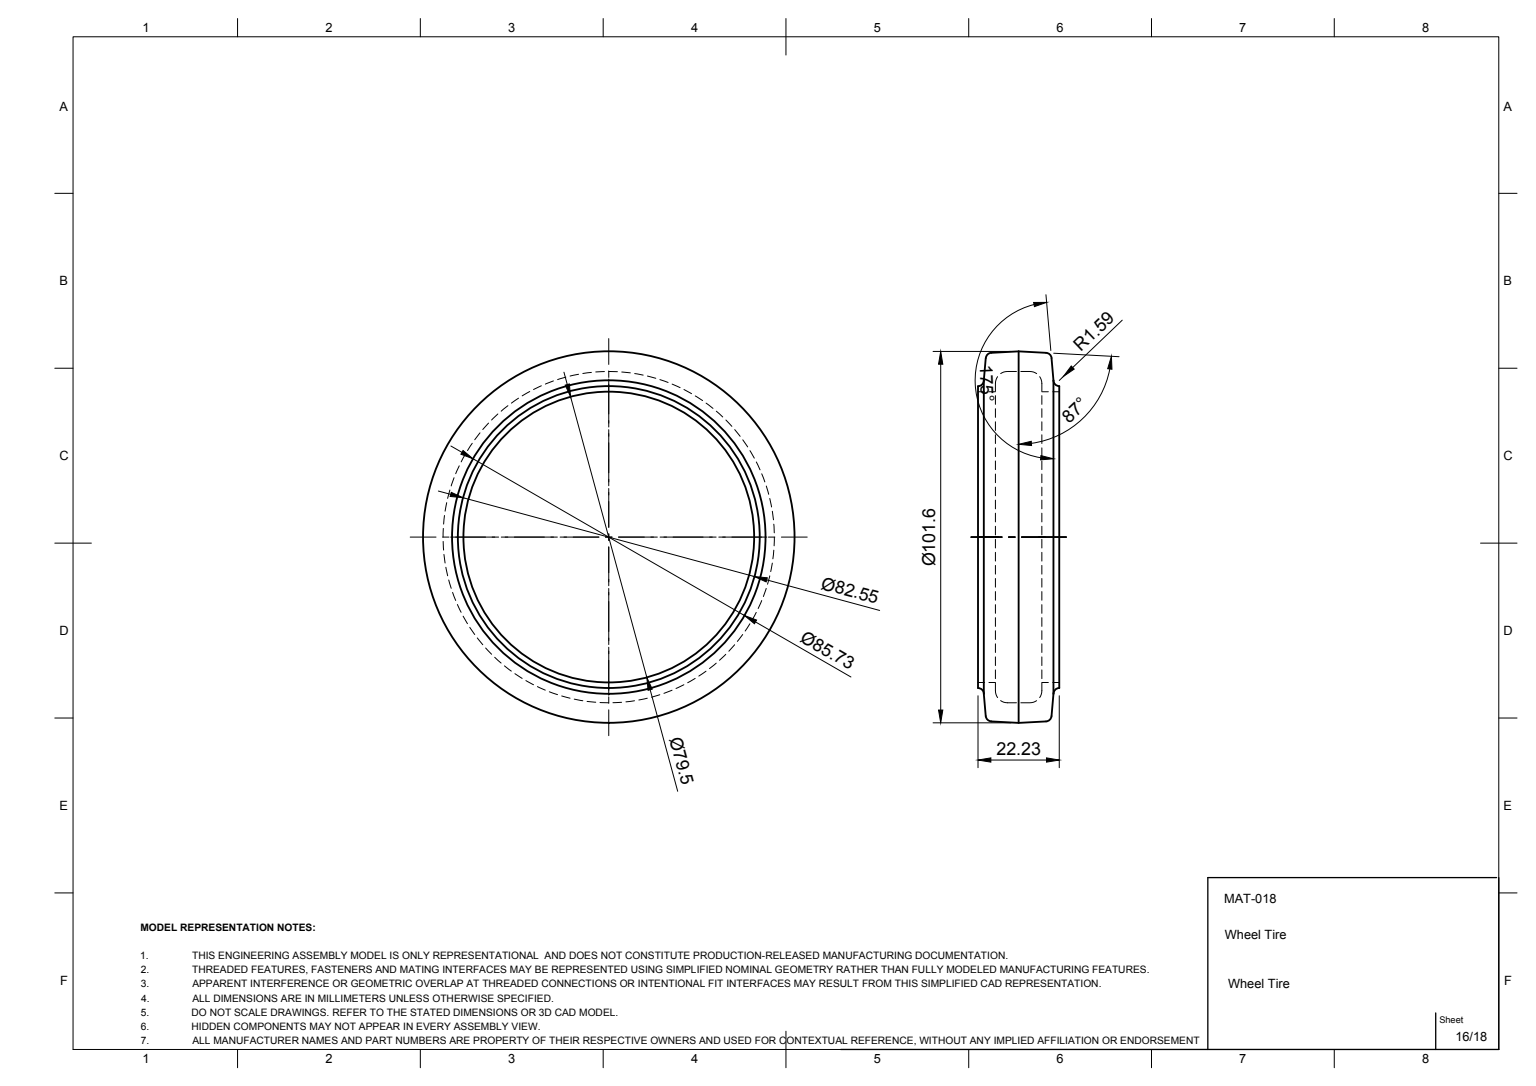
ISO-10303-21;
HEADER;
/* Generated by software containing ST-Developer
 * from STEP Tools, Inc. (www.steptools.com) 
 */

FILE_DESCRIPTION(
/* description */ ('STEP AP214'),
/* implementation_level */ '2;1');

FILE_NAME(
/* name */ 'Wheel Tire.step',
/* time_stamp */ '2026-11-14T06:16:09-08:00',
/* author */ (''),
/* organization */ (''),
/* preprocessor_version */ 'ST-DEVELOPER v20.2',
/* originating_system */ 'Autodesk Translation Framework v15.17.0.0',
/* authorisation */ '');

FILE_SCHEMA (('AUTOMOTIVE_DESIGN { 1 0 10303 214 3 1 1 }'));
ENDSEC;

DATA;
#10=MECHANICAL_DESIGN_GEOMETRIC_PRESENTATION_REPRESENTATION('',(#360),#18006);
#147=CONICAL_SURFACE('',#10793,42.8625,1.48352986419518);
#148=CONICAL_SURFACE('',#10800,50.4073015581831,0.0523598775598306);
#149=CONICAL_SURFACE('',#10803,50.8,0.0523598775598286);
#150=CONICAL_SURFACE('',#10808,48.9603369133721,1.48352986419518);
#262=TOROIDAL_SURFACE('',#10776,42.00525,3.302);
#263=TOROIDAL_SURFACE('',#10782,42.00525,3.302);
#264=TOROIDAL_SURFACE('',#10788,42.8625,1.5875);
#265=TOROIDAL_SURFACE('',#10796,48.8219771717602,1.5875);
#266=TOROIDAL_SURFACE('',#10805,48.8219771717602,1.5875);
#267=TOROIDAL_SURFACE('',#10810,42.8625,1.5875);
#328=SHAPE_REPRESENTATION_RELATIONSHIP('SRR','None',#18086,#344);
#344=ADVANCED_BREP_SHAPE_REPRESENTATION('',(#376),#18003);
#360=STYLED_ITEM('',(#18172),#376);
#376=MANIFOLD_SOLID_BREP('Body1',#9569);
#494=FACE_BOUND('',#2095,.T.);
#495=FACE_BOUND('',#2097,.T.);
#496=FACE_BOUND('',#2099,.T.);
#497=FACE_BOUND('',#2101,.T.);
#833=PLANE('',#10813);
#834=PLANE('',#10814);
#835=PLANE('',#10815);
#836=PLANE('',#10816);
#1390=FACE_OUTER_BOUND('',#2081,.T.);
#1391=FACE_OUTER_BOUND('',#2082,.T.);
#1392=FACE_OUTER_BOUND('',#2083,.T.);
#1393=FACE_OUTER_BOUND('',#2084,.T.);
#1394=FACE_OUTER_BOUND('',#2085,.T.);
#1395=FACE_OUTER_BOUND('',#2086,.T.);
#1396=FACE_OUTER_BOUND('',#2087,.T.);
#1397=FACE_OUTER_BOUND('',#2088,.T.);
#1398=FACE_OUTER_BOUND('',#2089,.T.);
#1399=FACE_OUTER_BOUND('',#2090,.T.);
#1400=FACE_OUTER_BOUND('',#2091,.T.);
#1401=FACE_OUTER_BOUND('',#2092,.T.);
#1402=FACE_OUTER_BOUND('',#2093,.T.);
#1403=FACE_OUTER_BOUND('',#2094,.T.);
#1404=FACE_OUTER_BOUND('',#2096,.T.);
#1405=FACE_OUTER_BOUND('',#2098,.T.);
#1406=FACE_OUTER_BOUND('',#2100,.T.);
#2081=EDGE_LOOP('',(#8706,#8707,#8708,#8709));
#2082=EDGE_LOOP('',(#8710,#8711,#8712,#8713));
#2083=EDGE_LOOP('',(#8714,#8715,#8716,#8717));
#2084=EDGE_LOOP('',(#8718,#8719,#8720,#8721));
#2085=EDGE_LOOP('',(#8722,#8723,#8724,#8725));
#2086=EDGE_LOOP('',(#8726,#8727,#8728,#8729,#8730));
#2087=EDGE_LOOP('',(#8731,#8732,#8733,#8734,#8735,#8736));
#2088=EDGE_LOOP('',(#8737,#8738,#8739,#8740,#8741,#8742));
#2089=EDGE_LOOP('',(#8743,#8744,#8745,#8746,#8747,#8748));
#2090=EDGE_LOOP('',(#8749,#8750,#8751,#8752,#8753));
#2091=EDGE_LOOP('',(#8754,#8755,#8756,#8757));
#2092=EDGE_LOOP('',(#8758,#8759,#8760,#8761));
#2093=EDGE_LOOP('',(#8762,#8763,#8764,#8765));
#2094=EDGE_LOOP('',(#8766));
#2095=EDGE_LOOP('',(#8767));
#2096=EDGE_LOOP('',(#8768));
#2097=EDGE_LOOP('',(#8769));
#2098=EDGE_LOOP('',(#8770));
#2099=EDGE_LOOP('',(#8771));
#2100=EDGE_LOOP('',(#8772));
#2101=EDGE_LOOP('',(#8773));
#2827=LINE('',#17838,#3551);
#2828=LINE('',#17848,#3552);
#2829=LINE('',#17858,#3553);
#2830=LINE('',#17872,#3554);
#2831=LINE('',#17884,#3555);
#2832=LINE('',#17888,#3556);
#2833=LINE('',#17896,#3557);
#3551=VECTOR('',#13624,39.751);
#3552=VECTOR('',#13637,45.30725);
#3553=VECTOR('',#13650,39.751);
#3554=VECTOR('',#13667,42.8625);
#3555=VECTOR('',#13682,50.4073015581831);
#3556=VECTOR('',#13687,50.8);
#3557=VECTOR('',#13698,48.9603369133721);
#3975=CIRCLE('',#10774,39.751);
#3976=CIRCLE('',#10775,39.751);
#3977=CIRCLE('',#10777,42.00525);
#3978=CIRCLE('',#10778,3.302);
#3979=CIRCLE('',#10779,45.30725);
#3980=CIRCLE('',#10781,45.30725);
#3981=CIRCLE('',#10783,3.302);
#3982=CIRCLE('',#10784,42.00525);
#3983=CIRCLE('',#10786,39.751);
#3984=CIRCLE('',#10787,39.751);
#3985=CIRCLE('',#10789,41.275);
#3986=CIRCLE('',#10790,1.5875);
#3987=CIRCLE('',#10791,42.8625);
#3988=CIRCLE('',#10792,42.8625);
#3989=CIRCLE('',#10794,48.9603369133721);
#3990=CIRCLE('',#10795,48.9603369133721);
#3991=CIRCLE('',#10797,1.5875);
#3992=CIRCLE('',#10798,50.4073015581831);
#3993=CIRCLE('',#10799,50.4073015581831);
#3994=CIRCLE('',#10801,50.8);
#3995=CIRCLE('',#10802,50.8);
#3996=CIRCLE('',#10804,50.4073015581831);
#3997=CIRCLE('',#10806,1.5875);
#3998=CIRCLE('',#10807,48.9603369133721);
#3999=CIRCLE('',#10809,42.8625);
#4000=CIRCLE('',#10811,1.5875);
#4001=CIRCLE('',#10812,41.275);
#4792=VERTEX_POINT('',#17835);
#4793=VERTEX_POINT('',#17837);
#4794=VERTEX_POINT('',#17841);
#4795=VERTEX_POINT('',#17843);
#4796=VERTEX_POINT('',#17847);
#4797=VERTEX_POINT('',#17851);
#4798=VERTEX_POINT('',#17855);
#4799=VERTEX_POINT('',#17857);
#4800=VERTEX_POINT('',#17861);
#4801=VERTEX_POINT('',#17863);
#4802=VERTEX_POINT('',#17865);
#4803=VERTEX_POINT('',#17869);
#4804=VERTEX_POINT('',#17870);
#4805=VERTEX_POINT('',#17875);
#4806=VERTEX_POINT('',#17877);
#4807=VERTEX_POINT('',#17881);
#4808=VERTEX_POINT('',#17882);
#4809=VERTEX_POINT('',#17887);
#4810=VERTEX_POINT('',#17891);
#4811=VERTEX_POINT('',#17895);
#4812=VERTEX_POINT('',#17899);
#6101=EDGE_CURVE('',#4792,#4792,#3975,.T.);
#6102=EDGE_CURVE('',#4792,#4793,#2827,.T.);
#6103=EDGE_CURVE('',#4793,#4793,#3976,.T.);
#6104=EDGE_CURVE('',#4794,#4794,#3977,.T.);
#6105=EDGE_CURVE('',#4794,#4795,#3978,.T.);
#6106=EDGE_CURVE('',#4795,#4795,#3979,.T.);
#6107=EDGE_CURVE('',#4795,#4796,#2828,.T.);
#6108=EDGE_CURVE('',#4796,#4796,#3980,.T.);
#6109=EDGE_CURVE('',#4796,#4797,#3981,.T.);
#6110=EDGE_CURVE('',#4797,#4797,#3982,.T.);
#6111=EDGE_CURVE('',#4798,#4798,#3983,.T.);
#6112=EDGE_CURVE('',#4798,#4799,#2829,.T.);
#6113=EDGE_CURVE('',#4799,#4799,#3984,.T.);
#6114=EDGE_CURVE('',#4800,#4800,#3985,.T.);
#6115=EDGE_CURVE('',#4800,#4801,#3986,.T.);
#6116=EDGE_CURVE('',#4801,#4802,#3987,.T.);
#6117=EDGE_CURVE('',#4802,#4801,#3988,.T.);
#6118=EDGE_CURVE('',#4803,#4804,#3989,.T.);
#6119=EDGE_CURVE('',#4804,#4802,#2830,.T.);
#6120=EDGE_CURVE('',#4804,#4803,#3990,.T.);
#6121=EDGE_CURVE('',#4803,#4805,#3991,.T.);
#6122=EDGE_CURVE('',#4805,#4806,#3992,.T.);
#6123=EDGE_CURVE('',#4806,#4805,#3993,.T.);
#6124=EDGE_CURVE('',#4807,#4808,#3994,.T.);
#6125=EDGE_CURVE('',#4808,#4806,#2831,.T.);
#6126=EDGE_CURVE('',#4808,#4807,#3995,.T.);
#6127=EDGE_CURVE('',#4807,#4809,#2832,.T.);
#6128=EDGE_CURVE('',#4809,#4809,#3996,.T.);
#6129=EDGE_CURVE('',#4809,#4810,#3997,.T.);
#6130=EDGE_CURVE('',#4810,#4810,#3998,.T.);
#6131=EDGE_CURVE('',#4810,#4811,#2833,.T.);
#6132=EDGE_CURVE('',#4811,#4811,#3999,.T.);
#6133=EDGE_CURVE('',#4811,#4812,#4000,.T.);
#6134=EDGE_CURVE('',#4812,#4812,#4001,.T.);
#8706=ORIENTED_EDGE('',*,*,#6101,.F.);
#8707=ORIENTED_EDGE('',*,*,#6102,.T.);
#8708=ORIENTED_EDGE('',*,*,#6103,.T.);
#8709=ORIENTED_EDGE('',*,*,#6102,.F.);
#8710=ORIENTED_EDGE('',*,*,#6104,.F.);
#8711=ORIENTED_EDGE('',*,*,#6105,.T.);
#8712=ORIENTED_EDGE('',*,*,#6106,.T.);
#8713=ORIENTED_EDGE('',*,*,#6105,.F.);
#8714=ORIENTED_EDGE('',*,*,#6106,.F.);
#8715=ORIENTED_EDGE('',*,*,#6107,.T.);
#8716=ORIENTED_EDGE('',*,*,#6108,.T.);
#8717=ORIENTED_EDGE('',*,*,#6107,.F.);
#8718=ORIENTED_EDGE('',*,*,#6108,.F.);
#8719=ORIENTED_EDGE('',*,*,#6109,.T.);
#8720=ORIENTED_EDGE('',*,*,#6110,.T.);
#8721=ORIENTED_EDGE('',*,*,#6109,.F.);
#8722=ORIENTED_EDGE('',*,*,#6111,.F.);
#8723=ORIENTED_EDGE('',*,*,#6112,.T.);
#8724=ORIENTED_EDGE('',*,*,#6113,.T.);
#8725=ORIENTED_EDGE('',*,*,#6112,.F.);
#8726=ORIENTED_EDGE('',*,*,#6114,.F.);
#8727=ORIENTED_EDGE('',*,*,#6115,.T.);
#8728=ORIENTED_EDGE('',*,*,#6116,.T.);
#8729=ORIENTED_EDGE('',*,*,#6117,.T.);
#8730=ORIENTED_EDGE('',*,*,#6115,.F.);
#8731=ORIENTED_EDGE('',*,*,#6118,.T.);
#8732=ORIENTED_EDGE('',*,*,#6119,.T.);
#8733=ORIENTED_EDGE('',*,*,#6116,.F.);
#8734=ORIENTED_EDGE('',*,*,#6117,.F.);
#8735=ORIENTED_EDGE('',*,*,#6119,.F.);
#8736=ORIENTED_EDGE('',*,*,#6120,.T.);
#8737=ORIENTED_EDGE('',*,*,#6118,.F.);
#8738=ORIENTED_EDGE('',*,*,#6121,.T.);
#8739=ORIENTED_EDGE('',*,*,#6122,.T.);
#8740=ORIENTED_EDGE('',*,*,#6123,.T.);
#8741=ORIENTED_EDGE('',*,*,#6121,.F.);
#8742=ORIENTED_EDGE('',*,*,#6120,.F.);
#8743=ORIENTED_EDGE('',*,*,#6124,.T.);
#8744=ORIENTED_EDGE('',*,*,#6125,.T.);
#8745=ORIENTED_EDGE('',*,*,#6122,.F.);
#8746=ORIENTED_EDGE('',*,*,#6123,.F.);
#8747=ORIENTED_EDGE('',*,*,#6125,.F.);
#8748=ORIENTED_EDGE('',*,*,#6126,.T.);
#8749=ORIENTED_EDGE('',*,*,#6124,.F.);
#8750=ORIENTED_EDGE('',*,*,#6127,.T.);
#8751=ORIENTED_EDGE('',*,*,#6128,.T.);
#8752=ORIENTED_EDGE('',*,*,#6127,.F.);
#8753=ORIENTED_EDGE('',*,*,#6126,.F.);
#8754=ORIENTED_EDGE('',*,*,#6128,.F.);
#8755=ORIENTED_EDGE('',*,*,#6129,.T.);
#8756=ORIENTED_EDGE('',*,*,#6130,.T.);
#8757=ORIENTED_EDGE('',*,*,#6129,.F.);
#8758=ORIENTED_EDGE('',*,*,#6130,.F.);
#8759=ORIENTED_EDGE('',*,*,#6131,.T.);
#8760=ORIENTED_EDGE('',*,*,#6132,.T.);
#8761=ORIENTED_EDGE('',*,*,#6131,.F.);
#8762=ORIENTED_EDGE('',*,*,#6132,.F.);
#8763=ORIENTED_EDGE('',*,*,#6133,.T.);
#8764=ORIENTED_EDGE('',*,*,#6134,.T.);
#8765=ORIENTED_EDGE('',*,*,#6133,.F.);
#8766=ORIENTED_EDGE('',*,*,#6114,.T.);
#8767=ORIENTED_EDGE('',*,*,#6113,.F.);
#8768=ORIENTED_EDGE('',*,*,#6110,.F.);
#8769=ORIENTED_EDGE('',*,*,#6111,.T.);
#8770=ORIENTED_EDGE('',*,*,#6104,.T.);
#8771=ORIENTED_EDGE('',*,*,#6103,.F.);
#8772=ORIENTED_EDGE('',*,*,#6134,.F.);
#8773=ORIENTED_EDGE('',*,*,#6101,.T.);
#8973=CYLINDRICAL_SURFACE('',#10773,39.751);
#8974=CYLINDRICAL_SURFACE('',#10780,45.30725);
#8975=CYLINDRICAL_SURFACE('',#10785,39.751);
#9529=ADVANCED_FACE('',(#1390),#8973,.F.);
#9530=ADVANCED_FACE('',(#1391),#262,.F.);
#9531=ADVANCED_FACE('',(#1392),#8974,.F.);
#9532=ADVANCED_FACE('',(#1393),#263,.F.);
#9533=ADVANCED_FACE('',(#1394),#8975,.F.);
#9534=ADVANCED_FACE('',(#1395),#264,.F.);
#9535=ADVANCED_FACE('',(#1396),#147,.T.);
#9536=ADVANCED_FACE('',(#1397),#265,.T.);
#9537=ADVANCED_FACE('',(#1398),#148,.T.);
#9538=ADVANCED_FACE('',(#1399),#149,.T.);
#9539=ADVANCED_FACE('',(#1400),#266,.T.);
#9540=ADVANCED_FACE('',(#1401),#150,.T.);
#9541=ADVANCED_FACE('',(#1402),#267,.F.);
#9542=ADVANCED_FACE('',(#1403,#494),#833,.T.);
#9543=ADVANCED_FACE('',(#1404,#495),#834,.T.);
#9544=ADVANCED_FACE('',(#1405,#496),#835,.T.);
#9545=ADVANCED_FACE('',(#1406,#497),#836,.T.);
#9569=CLOSED_SHELL('',(#9529,#9530,#9531,#9532,#9533,#9534,#9535,#9536,
#9537,#9538,#9539,#9540,#9541,#9542,#9543,#9544,#9545));
#10772=AXIS2_PLACEMENT_3D('',#17833,#13618,#13619);
#10773=AXIS2_PLACEMENT_3D('',#17834,#13620,#13621);
#10774=AXIS2_PLACEMENT_3D('',#17836,#13622,#13623);
#10775=AXIS2_PLACEMENT_3D('',#17839,#13625,#13626);
#10776=AXIS2_PLACEMENT_3D('',#17840,#13627,#13628);
#10777=AXIS2_PLACEMENT_3D('',#17842,#13629,#13630);
#10778=AXIS2_PLACEMENT_3D('',#17844,#13631,#13632);
#10779=AXIS2_PLACEMENT_3D('',#17845,#13633,#13634);
#10780=AXIS2_PLACEMENT_3D('',#17846,#13635,#13636);
#10781=AXIS2_PLACEMENT_3D('',#17849,#13638,#13639);
#10782=AXIS2_PLACEMENT_3D('',#17850,#13640,#13641);
#10783=AXIS2_PLACEMENT_3D('',#17852,#13642,#13643);
#10784=AXIS2_PLACEMENT_3D('',#17853,#13644,#13645);
#10785=AXIS2_PLACEMENT_3D('',#17854,#13646,#13647);
#10786=AXIS2_PLACEMENT_3D('',#17856,#13648,#13649);
#10787=AXIS2_PLACEMENT_3D('',#17859,#13651,#13652);
#10788=AXIS2_PLACEMENT_3D('',#17860,#13653,#13654);
#10789=AXIS2_PLACEMENT_3D('',#17862,#13655,#13656);
#10790=AXIS2_PLACEMENT_3D('',#17864,#13657,#13658);
#10791=AXIS2_PLACEMENT_3D('',#17866,#13659,#13660);
#10792=AXIS2_PLACEMENT_3D('',#17867,#13661,#13662);
#10793=AXIS2_PLACEMENT_3D('',#17868,#13663,#13664);
#10794=AXIS2_PLACEMENT_3D('',#17871,#13665,#13666);
#10795=AXIS2_PLACEMENT_3D('',#17873,#13668,#13669);
#10796=AXIS2_PLACEMENT_3D('',#17874,#13670,#13671);
#10797=AXIS2_PLACEMENT_3D('',#17876,#13672,#13673);
#10798=AXIS2_PLACEMENT_3D('',#17878,#13674,#13675);
#10799=AXIS2_PLACEMENT_3D('',#17879,#13676,#13677);
#10800=AXIS2_PLACEMENT_3D('',#17880,#13678,#13679);
#10801=AXIS2_PLACEMENT_3D('',#17883,#13680,#13681);
#10802=AXIS2_PLACEMENT_3D('',#17885,#13683,#13684);
#10803=AXIS2_PLACEMENT_3D('',#17886,#13685,#13686);
#10804=AXIS2_PLACEMENT_3D('',#17889,#13688,#13689);
#10805=AXIS2_PLACEMENT_3D('',#17890,#13690,#13691);
#10806=AXIS2_PLACEMENT_3D('',#17892,#13692,#13693);
#10807=AXIS2_PLACEMENT_3D('',#17893,#13694,#13695);
#10808=AXIS2_PLACEMENT_3D('',#17894,#13696,#13697);
#10809=AXIS2_PLACEMENT_3D('',#17897,#13699,#13700);
#10810=AXIS2_PLACEMENT_3D('',#17898,#13701,#13702);
#10811=AXIS2_PLACEMENT_3D('',#17900,#13703,#13704);
#10812=AXIS2_PLACEMENT_3D('',#17901,#13705,#13706);
#10813=AXIS2_PLACEMENT_3D('',#17902,#13707,#13708);
#10814=AXIS2_PLACEMENT_3D('',#17903,#13709,#13710);
#10815=AXIS2_PLACEMENT_3D('',#17904,#13711,#13712);
#10816=AXIS2_PLACEMENT_3D('',#17905,#13713,#13714);
#13618=DIRECTION('axis',(0.,0.,1.));
#13619=DIRECTION('refdir',(1.,0.,0.));
#13620=DIRECTION('center_axis',(0.,0.,-1.));
#13621=DIRECTION('ref_axis',(-1.,0.,0.));
#13622=DIRECTION('center_axis',(0.,0.,-1.));
#13623=DIRECTION('ref_axis',(-1.,0.,0.));
#13624=DIRECTION('',(0.,0.,-1.));
#13625=DIRECTION('center_axis',(0.,0.,-1.));
#13626=DIRECTION('ref_axis',(-1.,0.,0.));
#13627=DIRECTION('center_axis',(0.,0.,-1.));
#13628=DIRECTION('ref_axis',(-1.,0.,0.));
#13629=DIRECTION('center_axis',(0.,0.,-1.));
#13630=DIRECTION('ref_axis',(-1.,0.,0.));
#13631=DIRECTION('center_axis',(1.22464679914735E-16,1.,0.));
#13632=DIRECTION('ref_axis',(1.,-1.22464679914735E-16,0.));
#13633=DIRECTION('center_axis',(0.,0.,-1.));
#13634=DIRECTION('ref_axis',(-1.,0.,0.));
#13635=DIRECTION('center_axis',(0.,0.,-1.));
#13636=DIRECTION('ref_axis',(-1.,0.,0.));
#13637=DIRECTION('',(0.,0.,-1.));
#13638=DIRECTION('center_axis',(0.,0.,-1.));
#13639=DIRECTION('ref_axis',(-1.,0.,0.));
#13640=DIRECTION('center_axis',(0.,0.,-1.));
#13641=DIRECTION('ref_axis',(-1.,0.,0.));
#13642=DIRECTION('center_axis',(1.22464679914735E-16,1.,0.));
#13643=DIRECTION('ref_axis',(1.,-1.22464679914735E-16,0.));
#13644=DIRECTION('center_axis',(0.,0.,-1.));
#13645=DIRECTION('ref_axis',(-1.,0.,0.));
#13646=DIRECTION('center_axis',(0.,0.,-1.));
#13647=DIRECTION('ref_axis',(-1.,0.,0.));
#13648=DIRECTION('center_axis',(0.,0.,-1.));
#13649=DIRECTION('ref_axis',(-1.,0.,0.));
#13650=DIRECTION('',(0.,0.,-1.));
#13651=DIRECTION('center_axis',(0.,0.,-1.));
#13652=DIRECTION('ref_axis',(-1.,0.,0.));
#13653=DIRECTION('center_axis',(0.,0.,-1.));
#13654=DIRECTION('ref_axis',(-1.,0.,0.));
#13655=DIRECTION('center_axis',(0.,0.,-1.));
#13656=DIRECTION('ref_axis',(-1.,0.,0.));
#13657=DIRECTION('center_axis',(1.22464679914735E-16,1.,0.));
#13658=DIRECTION('ref_axis',(1.,-1.22464679914735E-16,0.));
#13659=DIRECTION('center_axis',(0.,0.,-1.));
#13660=DIRECTION('ref_axis',(-1.,0.,0.));
#13661=DIRECTION('center_axis',(0.,0.,-1.));
#13662=DIRECTION('ref_axis',(-1.,0.,0.));
#13663=DIRECTION('center_axis',(0.,0.,1.));
#13664=DIRECTION('ref_axis',(1.,0.,0.));
#13665=DIRECTION('center_axis',(0.,0.,-1.));
#13666=DIRECTION('ref_axis',(-1.,0.,0.));
#13667=DIRECTION('',(0.996194698091745,1.21998664834562E-16,-0.0871557427476583));
#13668=DIRECTION('center_axis',(0.,0.,-1.));
#13669=DIRECTION('ref_axis',(-1.,0.,0.));
#13670=DIRECTION('center_axis',(0.,0.,-1.));
#13671=DIRECTION('ref_axis',(-1.,0.,0.));
#13672=DIRECTION('center_axis',(-1.22464679914735E-16,-1.,0.));
#13673=DIRECTION('ref_axis',(1.,-1.22464679914735E-16,0.));
#13674=DIRECTION('center_axis',(0.,0.,-1.));
#13675=DIRECTION('ref_axis',(-1.,0.,0.));
#13676=DIRECTION('center_axis',(0.,0.,-1.));
#13677=DIRECTION('ref_axis',(-1.,0.,0.));
#13678=DIRECTION('center_axis',(0.,0.,1.));
#13679=DIRECTION('ref_axis',(1.,0.,0.));
#13680=DIRECTION('center_axis',(0.,0.,-1.));
#13681=DIRECTION('ref_axis',(-1.,0.,0.));
#13682=DIRECTION('',(0.0523359562429446,6.4093061293238E-18,-0.998629534754574));
#13683=DIRECTION('center_axis',(0.,0.,-1.));
#13684=DIRECTION('ref_axis',(-1.,0.,0.));
#13685=DIRECTION('center_axis',(0.,0.,-1.));
#13686=DIRECTION('ref_axis',(-1.,0.,0.));
#13687=DIRECTION('',(-0.0523359562429425,6.40930612932355E-18,0.998629534754574));
#13688=DIRECTION('center_axis',(0.,0.,-1.));
#13689=DIRECTION('ref_axis',(-1.,0.,0.));
#13690=DIRECTION('center_axis',(0.,0.,-1.));
#13691=DIRECTION('ref_axis',(-1.,0.,0.));
#13692=DIRECTION('center_axis',(-1.22464679914735E-16,-1.,0.));
#13693=DIRECTION('ref_axis',(1.,-1.22464679914735E-16,0.));
#13694=DIRECTION('center_axis',(0.,0.,-1.));
#13695=DIRECTION('ref_axis',(-1.,0.,0.));
#13696=DIRECTION('center_axis',(0.,0.,-1.));
#13697=DIRECTION('ref_axis',(-1.,0.,0.));
#13698=DIRECTION('',(-0.996194698091746,1.21998664834562E-16,0.0871557427476584));
#13699=DIRECTION('center_axis',(0.,0.,-1.));
#13700=DIRECTION('ref_axis',(-1.,0.,0.));
#13701=DIRECTION('center_axis',(0.,0.,-1.));
#13702=DIRECTION('ref_axis',(-1.,0.,0.));
#13703=DIRECTION('center_axis',(1.22464679914735E-16,1.,0.));
#13704=DIRECTION('ref_axis',(1.,-1.22464679914735E-16,0.));
#13705=DIRECTION('center_axis',(0.,0.,-1.));
#13706=DIRECTION('ref_axis',(-1.,0.,0.));
#13707=DIRECTION('center_axis',(0.,0.,-1.));
#13708=DIRECTION('ref_axis',(0.,-1.,0.));
#13709=DIRECTION('center_axis',(0.,0.,1.));
#13710=DIRECTION('ref_axis',(1.,0.,0.));
#13711=DIRECTION('center_axis',(0.,0.,-1.));
#13712=DIRECTION('ref_axis',(0.,-1.,0.));
#13713=DIRECTION('center_axis',(0.,0.,1.));
#13714=DIRECTION('ref_axis',(1.,0.,0.));
#17833=CARTESIAN_POINT('',(0.,0.,0.));
#17834=CARTESIAN_POINT('Origin',(-1.11022302462516E-12,0.,-11.1125));
#17835=CARTESIAN_POINT('',(39.7509999999989,-4.86809349129064E-15,11.1125));
#17836=CARTESIAN_POINT('Origin',(0.,0.,11.1125));
#17837=CARTESIAN_POINT('',(39.7509999999989,-4.86809349129064E-15,6.35000000000002));
#17838=CARTESIAN_POINT('',(39.7509999999989,-4.86809349129064E-15,-11.1125));
#17839=CARTESIAN_POINT('Origin',(-1.11022302462516E-12,0.,6.35000000000002));
#17840=CARTESIAN_POINT('Origin',(0.,0.,3.048));
#17841=CARTESIAN_POINT('',(42.0052499999989,-5.1441594959883E-15,6.35000000000002));
#17842=CARTESIAN_POINT('Origin',(-1.11022302462516E-12,0.,6.35000000000002));
#17843=CARTESIAN_POINT('',(45.30725,-5.54853786906689E-15,3.048));
#17844=CARTESIAN_POINT('Origin',(42.00525,-5.14415949598844E-15,3.048));
#17845=CARTESIAN_POINT('Origin',(0.,0.,3.048));
#17846=CARTESIAN_POINT('Origin',(-1.11022302462516E-12,0.,-11.1125));
#17847=CARTESIAN_POINT('',(45.3072499999989,-5.54853786906689E-15,-3.048));
#17848=CARTESIAN_POINT('',(45.3072499999989,-5.54853786906689E-15,-11.1125));
#17849=CARTESIAN_POINT('Origin',(-1.11022302462516E-12,0.,-3.048));
#17850=CARTESIAN_POINT('Origin',(-1.11022302462516E-12,0.,-3.048));
#17851=CARTESIAN_POINT('',(42.00525,-5.14415949598857E-15,-6.35000000000002));
#17852=CARTESIAN_POINT('Origin',(42.0052499999989,-5.14415949598844E-15,
-3.048));
#17853=CARTESIAN_POINT('Origin',(0.,0.,-6.35000000000002));
#17854=CARTESIAN_POINT('Origin',(-1.11022302462516E-12,0.,-11.1125));
#17855=CARTESIAN_POINT('',(39.7509999999989,-4.86809349129064E-15,-6.35000000000002));
#17856=CARTESIAN_POINT('Origin',(0.,0.,-6.35000000000002));
#17857=CARTESIAN_POINT('',(39.7509999999989,-4.86809349129064E-15,-11.1125));
#17858=CARTESIAN_POINT('',(39.7509999999989,-4.86809349129064E-15,-11.1125));
#17859=CARTESIAN_POINT('Origin',(-1.11022302462516E-12,0.,-11.1125));
#17860=CARTESIAN_POINT('Origin',(-1.11022302462516E-12,0.,-11.1125));
#17861=CARTESIAN_POINT('',(41.2749999999989,-5.0547296634807E-15,-11.1125));
#17862=CARTESIAN_POINT('Origin',(-1.11022302462516E-12,0.,-11.1125));
#17863=CARTESIAN_POINT('',(42.8625,-5.24914234284548E-15,-9.52500000000001));
#17864=CARTESIAN_POINT('Origin',(42.8624999999989,-5.24914234284534E-15,
-11.1125));
#17865=CARTESIAN_POINT('',(-42.8625,5.62252716572953E-15,-9.52500000000001));
#17866=CARTESIAN_POINT('Origin',(0.,0.,-9.52500000000001));
#17867=CARTESIAN_POINT('Origin',(0.,0.,-9.52500000000001));
#17868=CARTESIAN_POINT('Origin',(0.,0.,-9.52500000000001));
#17869=CARTESIAN_POINT('',(48.9603369133721,6.08451301965107E-15,-8.99150839805002));
#17870=CARTESIAN_POINT('',(-48.9603369133721,-5.99591198861371E-15,-8.99150839805003));
#17871=CARTESIAN_POINT('Origin',(0.,0.,-8.99150839805002));
#17872=CARTESIAN_POINT('',(-42.8625,-5.24914234284534E-15,-9.52500000000001));
#17873=CARTESIAN_POINT('Origin',(0.,0.,-8.99150839805002));
#17874=CARTESIAN_POINT('Origin',(0.,0.,-7.41004931482936));
#17875=CARTESIAN_POINT('',(50.4073015581831,-6.17311405068843E-15,-7.49313264536505));
#17876=CARTESIAN_POINT('Origin',(48.8219771717602,-5.97896780714413E-15,
-7.41004931482936));
#17877=CARTESIAN_POINT('',(-50.4073015581831,6.19715989517849E-15,-7.49313264536505));
#17878=CARTESIAN_POINT('Origin',(0.,0.,-7.49313264536505));
#17879=CARTESIAN_POINT('Origin',(0.,0.,-7.49313264536505));
#17880=CARTESIAN_POINT('Origin',(0.,0.,-7.49313264536505));
#17881=CARTESIAN_POINT('',(50.8,6.22120573966855E-15,0.));
#17882=CARTESIAN_POINT('',(-50.7999999999999,-6.22120573966855E-15,2.22044604925031E-15));
#17883=CARTESIAN_POINT('Origin',(0.,0.,0.));
#17884=CARTESIAN_POINT('',(-50.4073015581831,-6.17311405068843E-15,-7.49313264536505));
#17885=CARTESIAN_POINT('Origin',(0.,0.,0.));
#17886=CARTESIAN_POINT('Origin',(0.,0.,0.));
#17887=CARTESIAN_POINT('',(50.4073015581832,-6.17311405068844E-15,7.49313264536512));
#17888=CARTESIAN_POINT('',(50.8,-6.22120573966855E-15,0.));
#17889=CARTESIAN_POINT('Origin',(-1.11022302462516E-12,0.,7.49313264536505));
#17890=CARTESIAN_POINT('Origin',(-1.11022302462516E-12,0.,7.41004931482936));
#17891=CARTESIAN_POINT('',(48.960336913371,-5.99591198861371E-15,8.99150839805002));
#17892=CARTESIAN_POINT('Origin',(48.8219771717591,-5.97896780714413E-15,
7.41004931482936));
#17893=CARTESIAN_POINT('Origin',(-1.11022302462516E-12,0.,8.99150839805002));
#17894=CARTESIAN_POINT('Origin',(-1.11022302462516E-12,0.,8.99150839805002));
#17895=CARTESIAN_POINT('',(42.8624999999989,-5.24914234284534E-15,9.52499999999999));
#17896=CARTESIAN_POINT('',(48.960336913371,-5.99591198861371E-15,8.99150839805002));
#17897=CARTESIAN_POINT('Origin',(-1.11022302462516E-12,0.,9.52500000000001));
#17898=CARTESIAN_POINT('Origin',(0.,0.,11.1125));
#17899=CARTESIAN_POINT('',(41.275,-5.0547296634807E-15,11.1125));
#17900=CARTESIAN_POINT('Origin',(42.8625,-5.24914234284534E-15,11.1125));
#17901=CARTESIAN_POINT('Origin',(0.,0.,11.1125));
#17902=CARTESIAN_POINT('Origin',(-1.11022302462516E-12,39.751,-11.1125));
#17903=CARTESIAN_POINT('Origin',(0.,42.00525,-6.35000000000002));
#17904=CARTESIAN_POINT('Origin',(-1.11022302462516E-12,39.751,6.35000000000002));
#17905=CARTESIAN_POINT('Origin',(0.,41.275,11.1125));
#17983=UNCERTAINTY_MEASURE_WITH_UNIT(LENGTH_MEASURE(0.01),#18007,
'DISTANCE_ACCURACY_VALUE',
'Maximum model space distance between geometric entities at asserted c
onnectivities');
#17986=UNCERTAINTY_MEASURE_WITH_UNIT(LENGTH_MEASURE(0.01),#18007,
'DISTANCE_ACCURACY_VALUE',
'Maximum model space distance between geometric entities at asserted c
onnectivities');
#18003=(
GEOMETRIC_REPRESENTATION_CONTEXT(3)
GLOBAL_UNCERTAINTY_ASSIGNED_CONTEXT((#17983))
GLOBAL_UNIT_ASSIGNED_CONTEXT((#18007,#18009,#18010))
REPRESENTATION_CONTEXT('','3D')
);
#18006=(
GEOMETRIC_REPRESENTATION_CONTEXT(3)
GLOBAL_UNCERTAINTY_ASSIGNED_CONTEXT((#17986))
GLOBAL_UNIT_ASSIGNED_CONTEXT((#18007,#18009,#18010))
REPRESENTATION_CONTEXT('','3D')
);
#18007=(
LENGTH_UNIT()
NAMED_UNIT(*)
SI_UNIT(.MILLI.,.METRE.)
);
#18009=(
NAMED_UNIT(*)
PLANE_ANGLE_UNIT()
SI_UNIT($,.RADIAN.)
);
#18010=(
NAMED_UNIT(*)
SI_UNIT($,.STERADIAN.)
SOLID_ANGLE_UNIT()
);
#18027=SHAPE_DEFINITION_REPRESENTATION(#18046,#18086);
#18046=PRODUCT_DEFINITION_SHAPE('',$,#18106);
#18086=SHAPE_REPRESENTATION('',(#10772),#18003);
#18089=PRODUCT_DEFINITION_CONTEXT('part definition',#18148,'design');
#18106=PRODUCT_DEFINITION('Wheel Tire','Wheel Tire',#18125,#18089);
#18125=PRODUCT_DEFINITION_FORMATION('',$,#18166);
#18148=APPLICATION_CONTEXT(
'Core Data for Automotive Mechanical Design Process');
#18149=PRODUCT_CONTEXT('part definition',#18148,'mechanical');
#18166=PRODUCT('Wheel Tire','Wheel Tire',$,(#18149));
#18172=PRESENTATION_STYLE_ASSIGNMENT((#18176));
#18176=SURFACE_STYLE_USAGE(.BOTH.,#18180);
#18180=SURFACE_SIDE_STYLE('',(#18184));
#18184=SURFACE_STYLE_FILL_AREA(#18188);
#18188=FILL_AREA_STYLE('Opaque(97,158,199)',(#18192));
#18192=FILL_AREA_STYLE_COLOUR('Opaque(97,158,199)',#18196);
#18196=COLOUR_RGB('Opaque(97,158,199)',0.380392156862745,0.619607843137255,
0.780392156862745);
ENDSEC;
END-ISO-10303-21;
